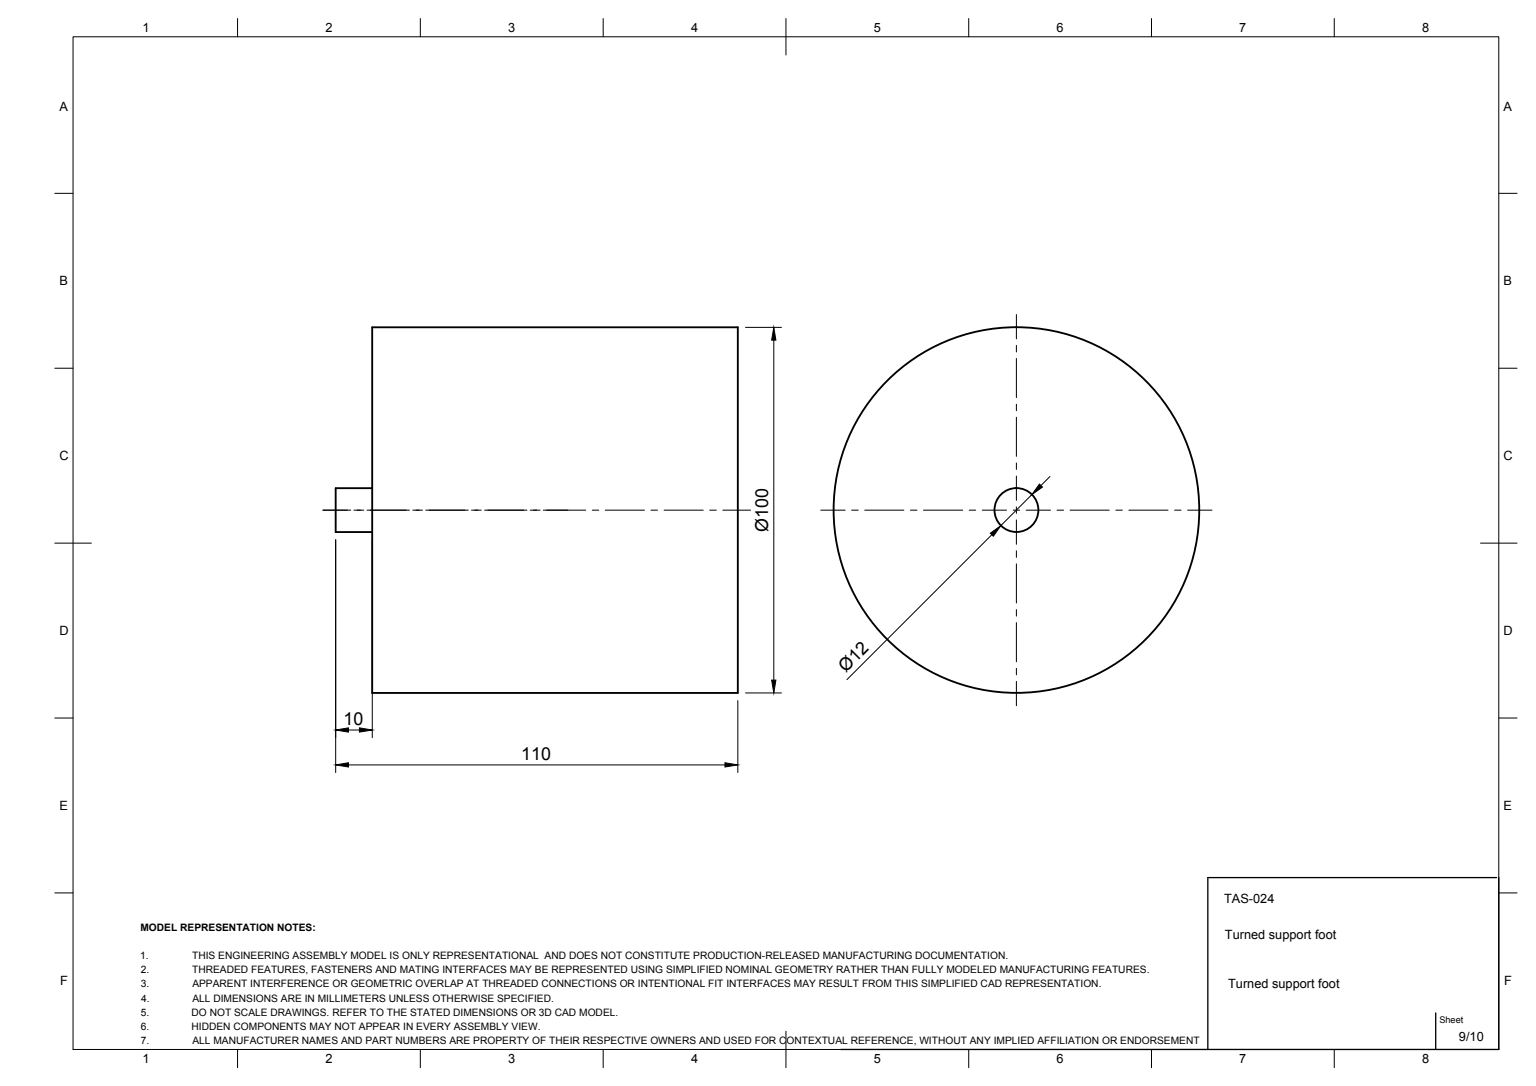
ISO-10303-21;
HEADER;
/* Generated by software containing ST-Developer
 * from STEP Tools, Inc. (www.steptools.com) 
 */

FILE_DESCRIPTION(
/* description */ (''),
/* implementation_level */ '2;1');

FILE_NAME(
/* name */ 'Turned support foot.step',
/* time_stamp */ '2026-11-15T17:53:25-08:00',
/* author */ (''),
/* organization */ (''),
/* preprocessor_version */ 'ST-DEVELOPER v20.2',
/* originating_system */ 'Autodesk Translation Framework v15.17.0.0',
/* authorisation */ '');

FILE_SCHEMA (('AUTOMOTIVE_DESIGN { 1 0 10303 214 3 1 1 }'));
ENDSEC;

DATA;
#10=MECHANICAL_DESIGN_GEOMETRIC_PRESENTATION_REPRESENTATION('',(#137),#2673);
#121=SHAPE_REPRESENTATION_RELATIONSHIP('SRR','None',#2729,#129);
#129=ADVANCED_BREP_SHAPE_REPRESENTATION('',(#145),#2671);
#137=STYLED_ITEM('',(#2778),#145);
#145=MANIFOLD_SOLID_BREP('Body1',#1523);
#159=FACE_BOUND('',#419,.T.);
#228=PLANE('',#1732);
#229=PLANE('',#1736);
#230=PLANE('',#1737);
#314=FACE_OUTER_BOUND('',#415,.T.);
#315=FACE_OUTER_BOUND('',#416,.T.);
#316=FACE_OUTER_BOUND('',#417,.T.);
#317=FACE_OUTER_BOUND('',#418,.T.);
#318=FACE_OUTER_BOUND('',#420,.T.);
#415=EDGE_LOOP('',(#1394,#1395,#1396,#1397));
#416=EDGE_LOOP('',(#1398));
#417=EDGE_LOOP('',(#1399,#1400,#1401,#1402));
#418=EDGE_LOOP('',(#1403));
#419=EDGE_LOOP('',(#1404));
#420=EDGE_LOOP('',(#1405));
#569=LINE('',#2608,#717);
#570=LINE('',#2615,#718);
#717=VECTOR('',#2149,0.6);
#718=VECTOR('',#2158,5.);
#746=CIRCLE('',#1730,0.6);
#747=CIRCLE('',#1731,0.6);
#748=CIRCLE('',#1734,5.);
#749=CIRCLE('',#1735,5.);
#866=VERTEX_POINT('',#2605);
#867=VERTEX_POINT('',#2607);
#868=VERTEX_POINT('',#2612);
#869=VERTEX_POINT('',#2614);
#1043=EDGE_CURVE('',#866,#866,#746,.T.);
#1044=EDGE_CURVE('',#866,#867,#569,.T.);
#1045=EDGE_CURVE('',#867,#867,#747,.T.);
#1046=EDGE_CURVE('',#868,#868,#748,.T.);
#1047=EDGE_CURVE('',#868,#869,#570,.T.);
#1048=EDGE_CURVE('',#869,#869,#749,.T.);
#1394=ORIENTED_EDGE('',*,*,#1043,.F.);
#1395=ORIENTED_EDGE('',*,*,#1044,.T.);
#1396=ORIENTED_EDGE('',*,*,#1045,.F.);
#1397=ORIENTED_EDGE('',*,*,#1044,.F.);
#1398=ORIENTED_EDGE('',*,*,#1043,.T.);
#1399=ORIENTED_EDGE('',*,*,#1046,.F.);
#1400=ORIENTED_EDGE('',*,*,#1047,.T.);
#1401=ORIENTED_EDGE('',*,*,#1048,.T.);
#1402=ORIENTED_EDGE('',*,*,#1047,.F.);
#1403=ORIENTED_EDGE('',*,*,#1046,.T.);
#1404=ORIENTED_EDGE('',*,*,#1045,.T.);
#1405=ORIENTED_EDGE('',*,*,#1048,.F.);
#1425=CYLINDRICAL_SURFACE('',#1729,0.6);
#1426=CYLINDRICAL_SURFACE('',#1733,5.);
#1509=ADVANCED_FACE('',(#314),#1425,.T.);
#1510=ADVANCED_FACE('',(#315),#228,.T.);
#1511=ADVANCED_FACE('',(#316),#1426,.T.);
#1512=ADVANCED_FACE('',(#317,#159),#229,.T.);
#1513=ADVANCED_FACE('',(#318),#230,.F.);
#1523=CLOSED_SHELL('',(#1509,#1510,#1511,#1512,#1513));
#1728=AXIS2_PLACEMENT_3D('',#2603,#2143,#2144);
#1729=AXIS2_PLACEMENT_3D('',#2604,#2145,#2146);
#1730=AXIS2_PLACEMENT_3D('',#2606,#2147,#2148);
#1731=AXIS2_PLACEMENT_3D('',#2609,#2150,#2151);
#1732=AXIS2_PLACEMENT_3D('',#2610,#2152,#2153);
#1733=AXIS2_PLACEMENT_3D('',#2611,#2154,#2155);
#1734=AXIS2_PLACEMENT_3D('',#2613,#2156,#2157);
#1735=AXIS2_PLACEMENT_3D('',#2616,#2159,#2160);
#1736=AXIS2_PLACEMENT_3D('',#2617,#2161,#2162);
#1737=AXIS2_PLACEMENT_3D('',#2618,#2163,#2164);
#2143=DIRECTION('axis',(0.,0.,1.));
#2144=DIRECTION('refdir',(1.,0.,0.));
#2145=DIRECTION('center_axis',(0.,0.,1.));
#2146=DIRECTION('ref_axis',(1.,0.,0.));
#2147=DIRECTION('center_axis',(0.,0.,1.));
#2148=DIRECTION('ref_axis',(1.,0.,0.));
#2149=DIRECTION('',(0.,0.,-1.));
#2150=DIRECTION('center_axis',(0.,0.,-1.));
#2151=DIRECTION('ref_axis',(1.,0.,0.));
#2152=DIRECTION('center_axis',(0.,0.,1.));
#2153=DIRECTION('ref_axis',(1.,0.,0.));
#2154=DIRECTION('center_axis',(0.,0.,1.));
#2155=DIRECTION('ref_axis',(1.,0.,0.));
#2156=DIRECTION('center_axis',(0.,0.,1.));
#2157=DIRECTION('ref_axis',(1.,0.,0.));
#2158=DIRECTION('',(0.,0.,-1.));
#2159=DIRECTION('center_axis',(0.,0.,1.));
#2160=DIRECTION('ref_axis',(1.,0.,0.));
#2161=DIRECTION('center_axis',(0.,0.,1.));
#2162=DIRECTION('ref_axis',(1.,0.,0.));
#2163=DIRECTION('center_axis',(0.,0.,1.));
#2164=DIRECTION('ref_axis',(1.,0.,0.));
#2603=CARTESIAN_POINT('',(0.,0.,0.));
#2604=CARTESIAN_POINT('Origin',(0.,0.,10.));
#2605=CARTESIAN_POINT('',(-0.6,-7.34788079488412E-17,11.));
#2606=CARTESIAN_POINT('Origin',(0.,0.,11.));
#2607=CARTESIAN_POINT('',(-0.6,-7.34788079488412E-17,10.));
#2608=CARTESIAN_POINT('',(-0.6,-7.34788079488412E-17,10.));
#2609=CARTESIAN_POINT('Origin',(0.,0.,10.));
#2610=CARTESIAN_POINT('Origin',(0.,0.,11.));
#2611=CARTESIAN_POINT('Origin',(0.,0.,0.));
#2612=CARTESIAN_POINT('',(-5.,-6.12323399573677E-16,10.));
#2613=CARTESIAN_POINT('Origin',(0.,0.,10.));
#2614=CARTESIAN_POINT('',(-5.,-6.12323399573677E-16,0.));
#2615=CARTESIAN_POINT('',(-5.,-6.12323399573677E-16,0.));
#2616=CARTESIAN_POINT('Origin',(0.,0.,0.));
#2617=CARTESIAN_POINT('Origin',(0.,0.,10.));
#2618=CARTESIAN_POINT('Origin',(0.,0.,0.));
#2661=UNCERTAINTY_MEASURE_WITH_UNIT(LENGTH_MEASURE(0.001),#2674,
'DISTANCE_ACCURACY_VALUE',
'Maximum model space distance between geometric entities at asserted c
onnectivities');
#2663=UNCERTAINTY_MEASURE_WITH_UNIT(LENGTH_MEASURE(0.001),#2674,
'DISTANCE_ACCURACY_VALUE',
'Maximum model space distance between geometric entities at asserted c
onnectivities');
#2671=(
GEOMETRIC_REPRESENTATION_CONTEXT(3)
GLOBAL_UNCERTAINTY_ASSIGNED_CONTEXT((#2661))
GLOBAL_UNIT_ASSIGNED_CONTEXT((#2674,#2676,#2677))
REPRESENTATION_CONTEXT('','3D')
);
#2673=(
GEOMETRIC_REPRESENTATION_CONTEXT(3)
GLOBAL_UNCERTAINTY_ASSIGNED_CONTEXT((#2663))
GLOBAL_UNIT_ASSIGNED_CONTEXT((#2674,#2676,#2677))
REPRESENTATION_CONTEXT('','3D')
);
#2674=(
LENGTH_UNIT()
NAMED_UNIT(*)
SI_UNIT(.CENTI.,.METRE.)
);
#2676=(
NAMED_UNIT(*)
PLANE_ANGLE_UNIT()
SI_UNIT($,.RADIAN.)
);
#2677=(
NAMED_UNIT(*)
SI_UNIT($,.STERADIAN.)
SOLID_ANGLE_UNIT()
);
#2685=SHAPE_DEFINITION_REPRESENTATION(#2694,#2729);
#2694=PRODUCT_DEFINITION_SHAPE('',$,#2739);
#2729=SHAPE_REPRESENTATION('',(#1728),#2671);
#2731=PRODUCT_DEFINITION_CONTEXT('part definition',#2760,'design');
#2739=PRODUCT_DEFINITION('Turned support foot','Turned support foot',#2748,
#2731);
#2748=PRODUCT_DEFINITION_FORMATION('',$,#2769);
#2760=APPLICATION_CONTEXT(
'Core Data for Automotive Mechanical Design Process');
#2761=PRODUCT_CONTEXT('part definition',#2760,'mechanical');
#2769=PRODUCT('Turned support foot','Turned support foot',$,(#2761));
#2778=PRESENTATION_STYLE_ASSIGNMENT((#2787));
#2787=SURFACE_STYLE_USAGE(.BOTH.,#2796);
#2796=SURFACE_SIDE_STYLE('',(#2805));
#2805=SURFACE_STYLE_FILL_AREA(#2814);
#2814=FILL_AREA_STYLE('Turned support foot finish',(#2823));
#2823=FILL_AREA_STYLE_COLOUR('Turned support foot finish',#2832);
#2832=COLOUR_RGB('Turned support foot finish',0.188235294117647,0.211764705882353,
0.247058823529412);
ENDSEC;
END-ISO-10303-21;
